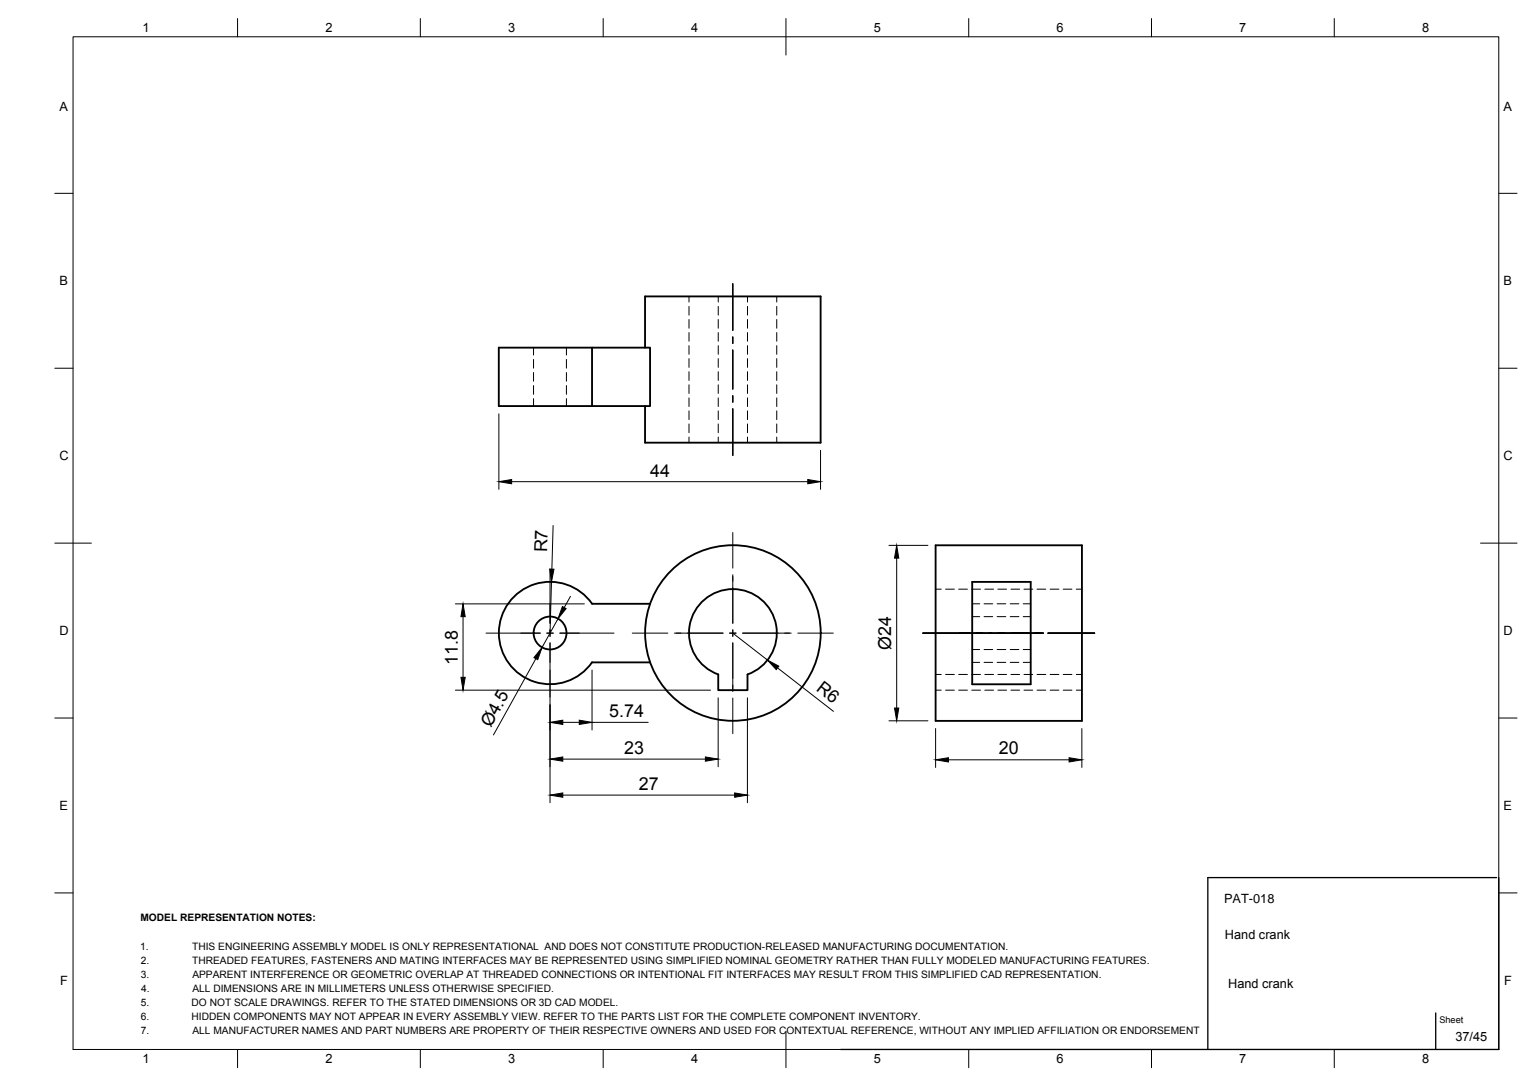
ISO-10303-21;
HEADER;
/* Generated by software containing ST-Developer
 * from STEP Tools, Inc. (www.steptools.com) 
 */

FILE_DESCRIPTION(
/* description */ ('Cam-driven reciprocating slide'),
/* implementation_level */ '2;1');

FILE_NAME(
/* name */ 'Hand crank.step',
/* time_stamp */ '2026-10-28T03:25:20-07:00',
/* author */ (''),
/* organization */ (''),
/* preprocessor_version */ 'ST-DEVELOPER v20.2',
/* originating_system */ 'Autodesk Translation Framework v15.17.0.0',
/* authorisation */ '');

FILE_SCHEMA (('AUTOMOTIVE_DESIGN { 1 0 10303 214 3 1 1 }'));
ENDSEC;

DATA;
#10=MECHANICAL_DESIGN_GEOMETRIC_PRESENTATION_REPRESENTATION('',(#457),#13277);
#376=SHAPE_REPRESENTATION_RELATIONSHIP('SRR','None',#13472,#413);
#413=ADVANCED_BREP_SHAPE_REPRESENTATION('',(#499),#13267);
#457=STYLED_ITEM('',(#13706),#499);
#499=MANIFOLD_SOLID_BREP('Body1',#6435);
#656=FACE_BOUND('',#1735,.T.);
#657=FACE_BOUND('',#1739,.T.);
#658=FACE_BOUND('',#1743,.T.);
#659=FACE_BOUND('',#1745,.T.);
#660=FACE_BOUND('',#1747,.T.);
#848=PLANE('',#7473);
#849=PLANE('',#7474);
#850=PLANE('',#7475);
#851=PLANE('',#7476);
#852=PLANE('',#7484);
#853=PLANE('',#7486);
#854=PLANE('',#7487);
#855=PLANE('',#7488);
#856=PLANE('',#7492);
#1202=FACE_OUTER_BOUND('',#1730,.T.);
#1203=FACE_OUTER_BOUND('',#1731,.T.);
#1204=FACE_OUTER_BOUND('',#1732,.T.);
#1205=FACE_OUTER_BOUND('',#1733,.T.);
#1206=FACE_OUTER_BOUND('',#1734,.T.);
#1207=FACE_OUTER_BOUND('',#1736,.T.);
#1208=FACE_OUTER_BOUND('',#1737,.T.);
#1209=FACE_OUTER_BOUND('',#1738,.T.);
#1210=FACE_OUTER_BOUND('',#1740,.T.);
#1211=FACE_OUTER_BOUND('',#1741,.T.);
#1212=FACE_OUTER_BOUND('',#1742,.T.);
#1213=FACE_OUTER_BOUND('',#1744,.T.);
#1214=FACE_OUTER_BOUND('',#1746,.T.);
#1730=EDGE_LOOP('',(#5582,#5583,#5584,#5585));
#1731=EDGE_LOOP('',(#5586,#5587,#5588,#5589));
#1732=EDGE_LOOP('',(#5590,#5591,#5592,#5593));
#1733=EDGE_LOOP('',(#5594,#5595,#5596,#5597));
#1734=EDGE_LOOP('',(#5598));
#1735=EDGE_LOOP('',(#5599,#5600,#5601,#5602));
#1736=EDGE_LOOP('',(#5603,#5604,#5605,#5606));
#1737=EDGE_LOOP('',(#5607,#5608,#5609,#5610));
#1738=EDGE_LOOP('',(#5611,#5612,#5613,#5614));
#1739=EDGE_LOOP('',(#5615));
#1740=EDGE_LOOP('',(#5616,#5617,#5618,#5619));
#1741=EDGE_LOOP('',(#5620,#5621,#5622,#5623));
#1742=EDGE_LOOP('',(#5624,#5625,#5626,#5627));
#1743=EDGE_LOOP('',(#5628));
#1744=EDGE_LOOP('',(#5629,#5630,#5631,#5632));
#1745=EDGE_LOOP('',(#5633,#5634,#5635,#5636));
#1746=EDGE_LOOP('',(#5637));
#1747=EDGE_LOOP('',(#5638,#5639,#5640,#5641));
#2165=LINE('',#12786,#2604);
#2166=LINE('',#12791,#2605);
#2167=LINE('',#12793,#2606);
#2168=LINE('',#12795,#2607);
#2169=LINE('',#12796,#2608);
#2170=LINE('',#12799,#2609);
#2171=LINE('',#12801,#2610);
#2172=LINE('',#12802,#2611);
#2173=LINE('',#12805,#2612);
#2174=LINE('',#12807,#2613);
#2175=LINE('',#12808,#2614);
#2176=LINE('',#12818,#2615);
#2177=LINE('',#12822,#2616);
#2178=LINE('',#12826,#2617);
#2179=LINE('',#12829,#2618);
#2180=LINE('',#12832,#2619);
#2181=LINE('',#12833,#2620);
#2182=LINE('',#12836,#2621);
#2183=LINE('',#12837,#2622);
#2184=LINE('',#12842,#2623);
#2604=VECTOR('',#9239,0.225);
#2605=VECTOR('',#9244,1.);
#2606=VECTOR('',#9245,1.);
#2607=VECTOR('',#9246,1.);
#2608=VECTOR('',#9247,1.);
#2609=VECTOR('',#9250,1.);
#2610=VECTOR('',#9251,1.);
#2611=VECTOR('',#9252,1.);
#2612=VECTOR('',#9255,1.);
#2613=VECTOR('',#9256,1.);
#2614=VECTOR('',#9257,1.);
#2615=VECTOR('',#9270,1.);
#2616=VECTOR('',#9273,1.);
#2617=VECTOR('',#9278,1.);
#2618=VECTOR('',#9281,1.);
#2619=VECTOR('',#9284,1.);
#2620=VECTOR('',#9285,1.);
#2621=VECTOR('',#9288,1.);
#2622=VECTOR('',#9289,1.);
#2623=VECTOR('',#9296,1.2);
#2987=CIRCLE('',#7471,0.225);
#2988=CIRCLE('',#7472,0.225);
#2989=CIRCLE('',#7477,1.2);
#2990=CIRCLE('',#7478,0.6);
#2991=CIRCLE('',#7480,0.6);
#2992=CIRCLE('',#7482,0.7);
#2993=CIRCLE('',#7483,0.7);
#2994=CIRCLE('',#7485,1.2);
#2995=CIRCLE('',#7489,1.2);
#2996=CIRCLE('',#7491,1.2);
#3456=VERTEX_POINT('',#12783);
#3457=VERTEX_POINT('',#12785);
#3458=VERTEX_POINT('',#12789);
#3459=VERTEX_POINT('',#12790);
#3460=VERTEX_POINT('',#12792);
#3461=VERTEX_POINT('',#12794);
#3462=VERTEX_POINT('',#12798);
#3463=VERTEX_POINT('',#12800);
#3464=VERTEX_POINT('',#12804);
#3465=VERTEX_POINT('',#12806);
#3466=VERTEX_POINT('',#12810);
#3467=VERTEX_POINT('',#12816);
#3468=VERTEX_POINT('',#12817);
#3469=VERTEX_POINT('',#12819);
#3470=VERTEX_POINT('',#12821);
#3471=VERTEX_POINT('',#12825);
#3472=VERTEX_POINT('',#12827);
#3473=VERTEX_POINT('',#12831);
#3474=VERTEX_POINT('',#12835);
#3475=VERTEX_POINT('',#12841);
#4181=EDGE_CURVE('',#3456,#3456,#2987,.T.);
#4182=EDGE_CURVE('',#3456,#3457,#2165,.T.);
#4183=EDGE_CURVE('',#3457,#3457,#2988,.T.);
#4184=EDGE_CURVE('',#3458,#3459,#2166,.T.);
#4185=EDGE_CURVE('',#3458,#3460,#2167,.T.);
#4186=EDGE_CURVE('',#3461,#3460,#2168,.T.);
#4187=EDGE_CURVE('',#3459,#3461,#2169,.T.);
#4188=EDGE_CURVE('',#3462,#3458,#2170,.T.);
#4189=EDGE_CURVE('',#3462,#3463,#2171,.T.);
#4190=EDGE_CURVE('',#3460,#3463,#2172,.T.);
#4191=EDGE_CURVE('',#3464,#3462,#2173,.T.);
#4192=EDGE_CURVE('',#3465,#3464,#2174,.T.);
#4193=EDGE_CURVE('',#3463,#3465,#2175,.T.);
#4194=EDGE_CURVE('',#3466,#3466,#2989,.T.);
#4195=EDGE_CURVE('',#3465,#3461,#2990,.T.);
#4196=EDGE_CURVE('',#3464,#3459,#2991,.T.);
#4197=EDGE_CURVE('',#3467,#3468,#2176,.T.);
#4198=EDGE_CURVE('',#3469,#3467,#2992,.T.);
#4199=EDGE_CURVE('',#3470,#3469,#2177,.T.);
#4200=EDGE_CURVE('',#3470,#3468,#2993,.T.);
#4201=EDGE_CURVE('',#3470,#3471,#2178,.T.);
#4202=EDGE_CURVE('',#3472,#3471,#2994,.T.);
#4203=EDGE_CURVE('',#3472,#3468,#2179,.T.);
#4204=EDGE_CURVE('',#3473,#3469,#2180,.T.);
#4205=EDGE_CURVE('',#3471,#3473,#2181,.T.);
#4206=EDGE_CURVE('',#3474,#3472,#2182,.T.);
#4207=EDGE_CURVE('',#3467,#3474,#2183,.T.);
#4208=EDGE_CURVE('',#3473,#3474,#2995,.T.);
#4209=EDGE_CURVE('',#3466,#3475,#2184,.T.);
#4210=EDGE_CURVE('',#3475,#3475,#2996,.T.);
#5582=ORIENTED_EDGE('',*,*,#4181,.F.);
#5583=ORIENTED_EDGE('',*,*,#4182,.T.);
#5584=ORIENTED_EDGE('',*,*,#4183,.F.);
#5585=ORIENTED_EDGE('',*,*,#4182,.F.);
#5586=ORIENTED_EDGE('',*,*,#4184,.F.);
#5587=ORIENTED_EDGE('',*,*,#4185,.T.);
#5588=ORIENTED_EDGE('',*,*,#4186,.F.);
#5589=ORIENTED_EDGE('',*,*,#4187,.F.);
#5590=ORIENTED_EDGE('',*,*,#4188,.F.);
#5591=ORIENTED_EDGE('',*,*,#4189,.T.);
#5592=ORIENTED_EDGE('',*,*,#4190,.F.);
#5593=ORIENTED_EDGE('',*,*,#4185,.F.);
#5594=ORIENTED_EDGE('',*,*,#4191,.F.);
#5595=ORIENTED_EDGE('',*,*,#4192,.F.);
#5596=ORIENTED_EDGE('',*,*,#4193,.F.);
#5597=ORIENTED_EDGE('',*,*,#4189,.F.);
#5598=ORIENTED_EDGE('',*,*,#4194,.T.);
#5599=ORIENTED_EDGE('',*,*,#4186,.T.);
#5600=ORIENTED_EDGE('',*,*,#4190,.T.);
#5601=ORIENTED_EDGE('',*,*,#4193,.T.);
#5602=ORIENTED_EDGE('',*,*,#4195,.T.);
#5603=ORIENTED_EDGE('',*,*,#4187,.T.);
#5604=ORIENTED_EDGE('',*,*,#4195,.F.);
#5605=ORIENTED_EDGE('',*,*,#4192,.T.);
#5606=ORIENTED_EDGE('',*,*,#4196,.T.);
#5607=ORIENTED_EDGE('',*,*,#4197,.F.);
#5608=ORIENTED_EDGE('',*,*,#4198,.F.);
#5609=ORIENTED_EDGE('',*,*,#4199,.F.);
#5610=ORIENTED_EDGE('',*,*,#4200,.T.);
#5611=ORIENTED_EDGE('',*,*,#4200,.F.);
#5612=ORIENTED_EDGE('',*,*,#4201,.T.);
#5613=ORIENTED_EDGE('',*,*,#4202,.F.);
#5614=ORIENTED_EDGE('',*,*,#4203,.T.);
#5615=ORIENTED_EDGE('',*,*,#4181,.T.);
#5616=ORIENTED_EDGE('',*,*,#4199,.T.);
#5617=ORIENTED_EDGE('',*,*,#4204,.F.);
#5618=ORIENTED_EDGE('',*,*,#4205,.F.);
#5619=ORIENTED_EDGE('',*,*,#4201,.F.);
#5620=ORIENTED_EDGE('',*,*,#4197,.T.);
#5621=ORIENTED_EDGE('',*,*,#4203,.F.);
#5622=ORIENTED_EDGE('',*,*,#4206,.F.);
#5623=ORIENTED_EDGE('',*,*,#4207,.F.);
#5624=ORIENTED_EDGE('',*,*,#4207,.T.);
#5625=ORIENTED_EDGE('',*,*,#4208,.F.);
#5626=ORIENTED_EDGE('',*,*,#4204,.T.);
#5627=ORIENTED_EDGE('',*,*,#4198,.T.);
#5628=ORIENTED_EDGE('',*,*,#4183,.T.);
#5629=ORIENTED_EDGE('',*,*,#4194,.F.);
#5630=ORIENTED_EDGE('',*,*,#4209,.T.);
#5631=ORIENTED_EDGE('',*,*,#4210,.T.);
#5632=ORIENTED_EDGE('',*,*,#4209,.F.);
#5633=ORIENTED_EDGE('',*,*,#4205,.T.);
#5634=ORIENTED_EDGE('',*,*,#4208,.T.);
#5635=ORIENTED_EDGE('',*,*,#4206,.T.);
#5636=ORIENTED_EDGE('',*,*,#4202,.T.);
#5637=ORIENTED_EDGE('',*,*,#4210,.F.);
#5638=ORIENTED_EDGE('',*,*,#4184,.T.);
#5639=ORIENTED_EDGE('',*,*,#4196,.F.);
#5640=ORIENTED_EDGE('',*,*,#4191,.T.);
#5641=ORIENTED_EDGE('',*,*,#4188,.T.);
#5998=CYLINDRICAL_SURFACE('',#7470,0.225);
#5999=CYLINDRICAL_SURFACE('',#7479,0.6);
#6000=CYLINDRICAL_SURFACE('',#7481,0.7);
#6001=CYLINDRICAL_SURFACE('',#7490,1.2);
#6320=ADVANCED_FACE('',(#1202),#5998,.F.);
#6321=ADVANCED_FACE('',(#1203),#848,.F.);
#6322=ADVANCED_FACE('',(#1204),#849,.F.);
#6323=ADVANCED_FACE('',(#1205),#850,.F.);
#6324=ADVANCED_FACE('',(#1206,#656),#851,.T.);
#6325=ADVANCED_FACE('',(#1207),#5999,.F.);
#6326=ADVANCED_FACE('',(#1208),#6000,.T.);
#6327=ADVANCED_FACE('',(#1209,#657),#852,.F.);
#6328=ADVANCED_FACE('',(#1210),#853,.T.);
#6329=ADVANCED_FACE('',(#1211),#854,.T.);
#6330=ADVANCED_FACE('',(#1212,#658),#855,.T.);
#6331=ADVANCED_FACE('',(#1213,#659),#6001,.T.);
#6332=ADVANCED_FACE('',(#1214,#660),#856,.F.);
#6435=CLOSED_SHELL('',(#6320,#6321,#6322,#6323,#6324,#6325,#6326,#6327,
#6328,#6329,#6330,#6331,#6332));
#7469=AXIS2_PLACEMENT_3D('',#12781,#9233,#9234);
#7470=AXIS2_PLACEMENT_3D('',#12782,#9235,#9236);
#7471=AXIS2_PLACEMENT_3D('',#12784,#9237,#9238);
#7472=AXIS2_PLACEMENT_3D('',#12787,#9240,#9241);
#7473=AXIS2_PLACEMENT_3D('',#12788,#9242,#9243);
#7474=AXIS2_PLACEMENT_3D('',#12797,#9248,#9249);
#7475=AXIS2_PLACEMENT_3D('',#12803,#9253,#9254);
#7476=AXIS2_PLACEMENT_3D('',#12809,#9258,#9259);
#7477=AXIS2_PLACEMENT_3D('',#12811,#9260,#9261);
#7478=AXIS2_PLACEMENT_3D('',#12812,#9262,#9263);
#7479=AXIS2_PLACEMENT_3D('',#12813,#9264,#9265);
#7480=AXIS2_PLACEMENT_3D('',#12814,#9266,#9267);
#7481=AXIS2_PLACEMENT_3D('',#12815,#9268,#9269);
#7482=AXIS2_PLACEMENT_3D('',#12820,#9271,#9272);
#7483=AXIS2_PLACEMENT_3D('',#12823,#9274,#9275);
#7484=AXIS2_PLACEMENT_3D('',#12824,#9276,#9277);
#7485=AXIS2_PLACEMENT_3D('',#12828,#9279,#9280);
#7486=AXIS2_PLACEMENT_3D('',#12830,#9282,#9283);
#7487=AXIS2_PLACEMENT_3D('',#12834,#9286,#9287);
#7488=AXIS2_PLACEMENT_3D('',#12838,#9290,#9291);
#7489=AXIS2_PLACEMENT_3D('',#12839,#9292,#9293);
#7490=AXIS2_PLACEMENT_3D('',#12840,#9294,#9295);
#7491=AXIS2_PLACEMENT_3D('',#12843,#9297,#9298);
#7492=AXIS2_PLACEMENT_3D('',#12844,#9299,#9300);
#9233=DIRECTION('axis',(0.,0.,1.));
#9234=DIRECTION('refdir',(1.,0.,0.));
#9235=DIRECTION('center_axis',(0.,1.,0.));
#9236=DIRECTION('ref_axis',(1.,0.,0.));
#9237=DIRECTION('center_axis',(0.,1.,0.));
#9238=DIRECTION('ref_axis',(1.,0.,0.));
#9239=DIRECTION('',(0.,1.,0.));
#9240=DIRECTION('center_axis',(0.,-1.,0.));
#9241=DIRECTION('ref_axis',(1.,0.,0.));
#9242=DIRECTION('center_axis',(-1.,0.,0.));
#9243=DIRECTION('ref_axis',(0.,0.,1.));
#9244=DIRECTION('',(0.,0.,1.));
#9245=DIRECTION('',(0.,1.,0.));
#9246=DIRECTION('',(0.,0.,-1.));
#9247=DIRECTION('',(0.,1.,0.));
#9248=DIRECTION('center_axis',(0.,0.,-1.));
#9249=DIRECTION('ref_axis',(-1.,0.,0.));
#9250=DIRECTION('',(-1.,0.,0.));
#9251=DIRECTION('',(0.,1.,0.));
#9252=DIRECTION('',(1.,0.,0.));
#9253=DIRECTION('center_axis',(1.,0.,0.));
#9254=DIRECTION('ref_axis',(0.,0.,-1.));
#9255=DIRECTION('',(0.,0.,-1.));
#9256=DIRECTION('',(0.,-1.,0.));
#9257=DIRECTION('',(0.,0.,1.));
#9258=DIRECTION('center_axis',(0.,1.,0.));
#9259=DIRECTION('ref_axis',(1.,0.,0.));
#9260=DIRECTION('center_axis',(0.,1.,0.));
#9261=DIRECTION('ref_axis',(1.,0.,0.));
#9262=DIRECTION('center_axis',(0.,-1.,0.));
#9263=DIRECTION('ref_axis',(1.,0.,0.));
#9264=DIRECTION('center_axis',(0.,1.,0.));
#9265=DIRECTION('ref_axis',(-1.83697019872103E-16,0.,1.));
#9266=DIRECTION('center_axis',(0.,-1.,0.));
#9267=DIRECTION('ref_axis',(1.,0.,0.));
#9268=DIRECTION('center_axis',(0.,1.,0.));
#9269=DIRECTION('ref_axis',(1.,0.,0.));
#9270=DIRECTION('',(0.,-1.,0.));
#9271=DIRECTION('center_axis',(0.,1.,0.));
#9272=DIRECTION('ref_axis',(1.,0.,0.));
#9273=DIRECTION('',(0.,1.,0.));
#9274=DIRECTION('center_axis',(0.,1.,0.));
#9275=DIRECTION('ref_axis',(1.,0.,0.));
#9276=DIRECTION('center_axis',(0.,1.,0.));
#9277=DIRECTION('ref_axis',(1.,0.,0.));
#9278=DIRECTION('',(-1.,0.,0.));
#9279=DIRECTION('center_axis',(0.,-1.,0.));
#9280=DIRECTION('ref_axis',(1.,0.,0.));
#9281=DIRECTION('',(1.,0.,0.));
#9282=DIRECTION('center_axis',(0.,0.,1.));
#9283=DIRECTION('ref_axis',(1.,0.,0.));
#9284=DIRECTION('',(1.,0.,0.));
#9285=DIRECTION('',(0.,1.,0.));
#9286=DIRECTION('center_axis',(0.,0.,-1.));
#9287=DIRECTION('ref_axis',(-1.,0.,0.));
#9288=DIRECTION('',(0.,-1.,0.));
#9289=DIRECTION('',(-1.,0.,0.));
#9290=DIRECTION('center_axis',(0.,1.,0.));
#9291=DIRECTION('ref_axis',(0.,0.,1.));
#9292=DIRECTION('center_axis',(0.,1.,0.));
#9293=DIRECTION('ref_axis',(1.,0.,0.));
#9294=DIRECTION('center_axis',(0.,1.,0.));
#9295=DIRECTION('ref_axis',(1.,0.,0.));
#9296=DIRECTION('',(0.,-1.,0.));
#9297=DIRECTION('center_axis',(0.,1.,0.));
#9298=DIRECTION('ref_axis',(1.,0.,0.));
#9299=DIRECTION('center_axis',(0.,1.,0.));
#9300=DIRECTION('ref_axis',(1.,0.,0.));
#12781=CARTESIAN_POINT('',(0.,0.,0.));
#12782=CARTESIAN_POINT('Origin',(2.5,4.9,4.));
#12783=CARTESIAN_POINT('',(2.275,5.,4.));
#12784=CARTESIAN_POINT('Origin',(2.5,5.,4.));
#12785=CARTESIAN_POINT('',(2.275,5.8,4.));
#12786=CARTESIAN_POINT('',(2.275,4.9,4.));
#12787=CARTESIAN_POINT('Origin',(2.5,5.8,4.));
#12788=CARTESIAN_POINT('Origin',(-0.2,4.4,3.22));
#12789=CARTESIAN_POINT('',(-0.2,4.5,3.22));
#12790=CARTESIAN_POINT('',(-0.2,4.5,3.43431457505076));
#12791=CARTESIAN_POINT('',(-0.2,4.5,3.61));
#12792=CARTESIAN_POINT('',(-0.2,6.5,3.22));
#12793=CARTESIAN_POINT('',(-0.2,4.4,3.22));
#12794=CARTESIAN_POINT('',(-0.2,6.5,3.43431457505076));
#12795=CARTESIAN_POINT('',(-0.2,6.5,3.61));
#12796=CARTESIAN_POINT('',(-0.2,4.5,3.43431457505076));
#12797=CARTESIAN_POINT('Origin',(0.2,4.4,3.22));
#12798=CARTESIAN_POINT('',(0.2,4.5,3.22));
#12799=CARTESIAN_POINT('',(0.1,4.5,3.22));
#12800=CARTESIAN_POINT('',(0.2,6.5,3.22));
#12801=CARTESIAN_POINT('',(0.2,4.4,3.22));
#12802=CARTESIAN_POINT('',(0.1,6.5,3.22));
#12803=CARTESIAN_POINT('Origin',(0.2,4.4,4.));
#12804=CARTESIAN_POINT('',(0.2,4.5,3.43431457505076));
#12805=CARTESIAN_POINT('',(0.2,4.5,4.));
#12806=CARTESIAN_POINT('',(0.2,6.5,3.43431457505076));
#12807=CARTESIAN_POINT('',(0.2,4.5,3.43431457505076));
#12808=CARTESIAN_POINT('',(0.2,6.5,4.));
#12809=CARTESIAN_POINT('Origin',(0.,6.5,4.));
#12810=CARTESIAN_POINT('',(-1.2,6.5,4.));
#12811=CARTESIAN_POINT('Origin',(0.,6.5,4.));
#12812=CARTESIAN_POINT('Origin',(0.,6.5,4.));
#12813=CARTESIAN_POINT('Origin',(0.,4.5,4.));
#12814=CARTESIAN_POINT('Origin',(0.,4.5,4.));
#12815=CARTESIAN_POINT('Origin',(2.5,5.,4.));
#12816=CARTESIAN_POINT('',(1.9255437353462,5.8,3.6));
#12817=CARTESIAN_POINT('',(1.9255437353462,5.,3.6));
#12818=CARTESIAN_POINT('',(1.9255437353462,5.,3.6));
#12819=CARTESIAN_POINT('',(1.9255437353462,5.8,4.4));
#12820=CARTESIAN_POINT('Origin',(2.5,5.8,4.));
#12821=CARTESIAN_POINT('',(1.9255437353462,5.,4.4));
#12822=CARTESIAN_POINT('',(1.9255437353462,5.,4.4));
#12823=CARTESIAN_POINT('Origin',(2.5,5.,4.));
#12824=CARTESIAN_POINT('Origin',(1.25,5.,4.));
#12825=CARTESIAN_POINT('',(1.13137084989848,5.,4.4));
#12826=CARTESIAN_POINT('',(2.5,5.,4.4));
#12827=CARTESIAN_POINT('',(1.13137084989848,5.,3.6));
#12828=CARTESIAN_POINT('Origin',(0.,5.,4.));
#12829=CARTESIAN_POINT('',(0.,5.,3.6));
#12830=CARTESIAN_POINT('Origin',(0.,5.,4.4));
#12831=CARTESIAN_POINT('',(1.13137084989848,5.8,4.4));
#12832=CARTESIAN_POINT('',(2.5,5.8,4.4));
#12833=CARTESIAN_POINT('',(1.13137084989848,4.5,4.4));
#12834=CARTESIAN_POINT('Origin',(2.5,5.,3.6));
#12835=CARTESIAN_POINT('',(1.13137084989848,5.8,3.6));
#12836=CARTESIAN_POINT('',(1.13137084989848,4.5,3.6));
#12837=CARTESIAN_POINT('',(0.,5.8,3.6));
#12838=CARTESIAN_POINT('Origin',(1.25,5.8,4.));
#12839=CARTESIAN_POINT('Origin',(0.,5.8,4.));
#12840=CARTESIAN_POINT('Origin',(0.,4.5,4.));
#12841=CARTESIAN_POINT('',(-1.2,4.5,4.));
#12842=CARTESIAN_POINT('',(-1.2,4.5,4.));
#12843=CARTESIAN_POINT('Origin',(0.,4.5,4.));
#12844=CARTESIAN_POINT('Origin',(0.,4.5,4.));
#13223=UNCERTAINTY_MEASURE_WITH_UNIT(LENGTH_MEASURE(0.001),#13278,
'DISTANCE_ACCURACY_VALUE',
'Maximum model space distance between geometric entities at asserted c
onnectivities');
#13233=UNCERTAINTY_MEASURE_WITH_UNIT(LENGTH_MEASURE(0.001),#13278,
'DISTANCE_ACCURACY_VALUE',
'Maximum model space distance between geometric entities at asserted c
onnectivities');
#13267=(
GEOMETRIC_REPRESENTATION_CONTEXT(3)
GLOBAL_UNCERTAINTY_ASSIGNED_CONTEXT((#13223))
GLOBAL_UNIT_ASSIGNED_CONTEXT((#13278,#13280,#13281))
REPRESENTATION_CONTEXT('','3D')
);
#13277=(
GEOMETRIC_REPRESENTATION_CONTEXT(3)
GLOBAL_UNCERTAINTY_ASSIGNED_CONTEXT((#13233))
GLOBAL_UNIT_ASSIGNED_CONTEXT((#13278,#13280,#13281))
REPRESENTATION_CONTEXT('','3D')
);
#13278=(
LENGTH_UNIT()
NAMED_UNIT(*)
SI_UNIT(.CENTI.,.METRE.)
);
#13280=(
NAMED_UNIT(*)
PLANE_ANGLE_UNIT()
SI_UNIT($,.RADIAN.)
);
#13281=(
NAMED_UNIT(*)
SI_UNIT($,.STERADIAN.)
SOLID_ANGLE_UNIT()
);
#13315=SHAPE_DEFINITION_REPRESENTATION(#13365,#13472);
#13365=PRODUCT_DEFINITION_SHAPE('',$,#13516);
#13472=SHAPE_REPRESENTATION('',(#7469),#13267);
#13482=PRODUCT_DEFINITION_CONTEXT('part definition',#13613,'design');
#13516=PRODUCT_DEFINITION('Hand crank','Hand crank',#13559,#13482);
#13559=PRODUCT_DEFINITION_FORMATION('',$,#13648);
#13613=APPLICATION_CONTEXT(
'Core Data for Automotive Mechanical Design Process');
#13614=PRODUCT_CONTEXT('part definition',#13613,'mechanical');
#13648=PRODUCT('Hand crank','Hand crank','Hand crank',(#13614));
#13700=COLOUR_RGB('Light Blue',0.38,0.62,0.78);
#13701=FILL_AREA_STYLE_COLOUR('',#13700);
#13702=FILL_AREA_STYLE('',(#13701));
#13703=SURFACE_STYLE_FILL_AREA(#13702);
#13704=SURFACE_SIDE_STYLE('',(#13703));
#13705=SURFACE_STYLE_USAGE(.BOTH.,#13704);
#13706=PRESENTATION_STYLE_ASSIGNMENT((#13705));
ENDSEC;
END-ISO-10303-21;
